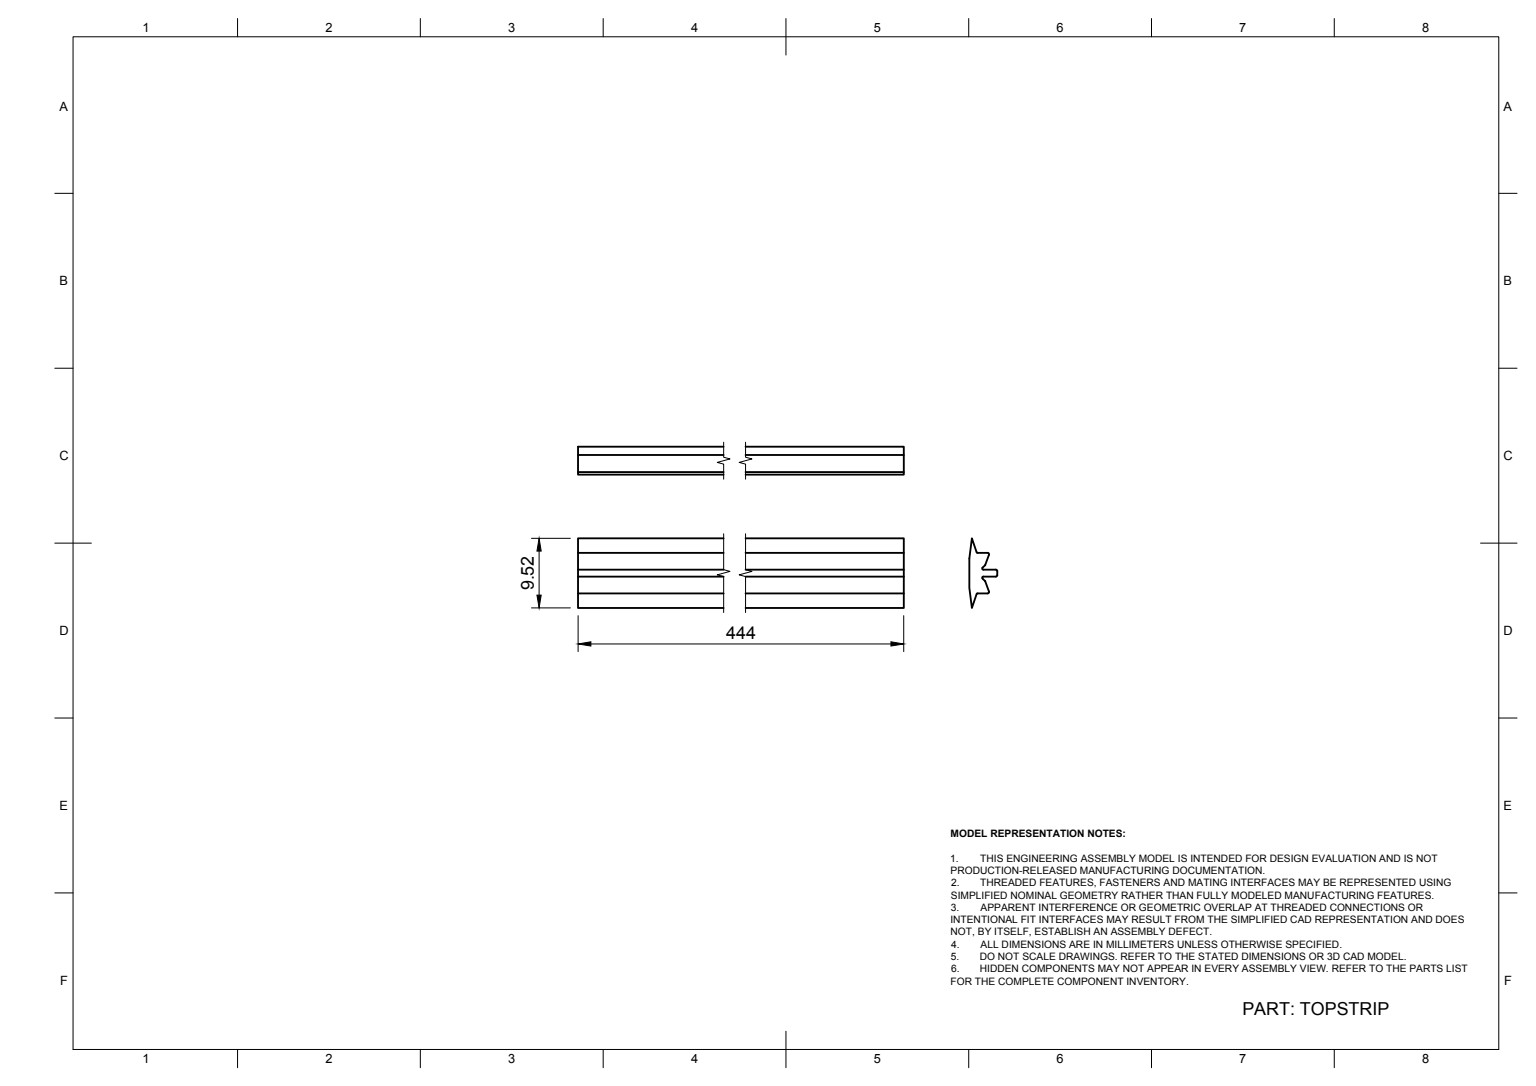
ISO-10303-21;
HEADER;
/* Generated by software containing ST-Developer
 * from STEP Tools, Inc. (www.steptools.com) 
 */

FILE_DESCRIPTION(
/* description */ (''),
/* implementation_level */ '2;1');

FILE_NAME(
/* name */ 'TopStrip.step',
/* time_stamp */ '2026-10-05T11:01:41-07:00',
/* author */ (''),
/* organization */ (''),
/* preprocessor_version */ 'ST-DEVELOPER v20.2',
/* originating_system */ 'Autodesk Translation Framework v15.15.0.0',
/* authorisation */ '');

FILE_SCHEMA (('AUTOMOTIVE_DESIGN { 1 0 10303 214 3 1 1 }'));
ENDSEC;

DATA;
#10=MECHANICAL_DESIGN_GEOMETRIC_PRESENTATION_REPRESENTATION('',(#2137),#215609);
#2119=SHAPE_REPRESENTATION_RELATIONSHIP('SRR','None',#215644,#2128);
#2128=ADVANCED_BREP_SHAPE_REPRESENTATION('',(#2146),#215600);
#2137=STYLED_ITEM('',(#215698),#2146);
#2146=MANIFOLD_SOLID_BREP('Body1',#28080);
#2155=CYLINDRICAL_SURFACE('',#28193,0.127);
#2156=CYLINDRICAL_SURFACE('',#28196,0.202999999999999);
#2157=CYLINDRICAL_SURFACE('',#28199,0.127000000000001);
#2158=CYLINDRICAL_SURFACE('',#28202,0.159000000000001);
#2159=CYLINDRICAL_SURFACE('',#28205,0.203000000000001);
#2160=CYLINDRICAL_SURFACE('',#28209,0.203);
#2161=CYLINDRICAL_SURFACE('',#28212,0.159000000000001);
#2162=CYLINDRICAL_SURFACE('',#28215,0.127000000000001);
#2163=CYLINDRICAL_SURFACE('',#28218,0.203);
#2164=CYLINDRICAL_SURFACE('',#28221,0.126999999999999);
#2964=FACE_OUTER_BOUND('',#4277,.T.);
#2965=FACE_OUTER_BOUND('',#4278,.T.);
#2966=FACE_OUTER_BOUND('',#4279,.T.);
#2967=FACE_OUTER_BOUND('',#4280,.T.);
#2968=FACE_OUTER_BOUND('',#4281,.T.);
#2969=FACE_OUTER_BOUND('',#4282,.T.);
#2970=FACE_OUTER_BOUND('',#4283,.T.);
#2971=FACE_OUTER_BOUND('',#4284,.T.);
#2972=FACE_OUTER_BOUND('',#4285,.T.);
#2973=FACE_OUTER_BOUND('',#4286,.T.);
#2974=FACE_OUTER_BOUND('',#4287,.T.);
#2975=FACE_OUTER_BOUND('',#4288,.T.);
#2976=FACE_OUTER_BOUND('',#4289,.T.);
#2977=FACE_OUTER_BOUND('',#4290,.T.);
#2978=FACE_OUTER_BOUND('',#4291,.T.);
#2979=FACE_OUTER_BOUND('',#4292,.T.);
#2980=FACE_OUTER_BOUND('',#4293,.T.);
#2981=FACE_OUTER_BOUND('',#4294,.T.);
#2982=FACE_OUTER_BOUND('',#4295,.T.);
#2983=FACE_OUTER_BOUND('',#4296,.T.);
#2984=FACE_OUTER_BOUND('',#4297,.T.);
#2985=FACE_OUTER_BOUND('',#4298,.T.);
#2986=FACE_OUTER_BOUND('',#4299,.T.);
#2987=FACE_OUTER_BOUND('',#4300,.T.);
#2988=FACE_OUTER_BOUND('',#4301,.T.);
#2989=FACE_OUTER_BOUND('',#4302,.T.);
#2990=FACE_OUTER_BOUND('',#4303,.T.);
#4277=EDGE_LOOP('',(#17529,#17530,#17531,#17532,#17533,#17534,#17535,#17536,
#17537,#17538,#17539,#17540,#17541,#17542,#17543,#17544,#17545,#17546,#17547,
#17548,#17549,#17550,#17551,#17552,#17553));
#4278=EDGE_LOOP('',(#17554,#17555,#17556,#17557));
#4279=EDGE_LOOP('',(#17558,#17559,#17560,#17561));
#4280=EDGE_LOOP('',(#17562,#17563,#17564,#17565));
#4281=EDGE_LOOP('',(#17566,#17567,#17568,#17569));
#4282=EDGE_LOOP('',(#17570,#17571,#17572,#17573));
#4283=EDGE_LOOP('',(#17574,#17575,#17576,#17577));
#4284=EDGE_LOOP('',(#17578,#17579,#17580,#17581));
#4285=EDGE_LOOP('',(#17582,#17583,#17584,#17585));
#4286=EDGE_LOOP('',(#17586,#17587,#17588,#17589));
#4287=EDGE_LOOP('',(#17590,#17591,#17592,#17593));
#4288=EDGE_LOOP('',(#17594,#17595,#17596,#17597));
#4289=EDGE_LOOP('',(#17598,#17599,#17600,#17601));
#4290=EDGE_LOOP('',(#17602,#17603,#17604,#17605));
#4291=EDGE_LOOP('',(#17606,#17607,#17608,#17609));
#4292=EDGE_LOOP('',(#17610,#17611,#17612,#17613));
#4293=EDGE_LOOP('',(#17614,#17615,#17616,#17617));
#4294=EDGE_LOOP('',(#17618,#17619,#17620,#17621));
#4295=EDGE_LOOP('',(#17622,#17623,#17624,#17625));
#4296=EDGE_LOOP('',(#17626,#17627,#17628,#17629));
#4297=EDGE_LOOP('',(#17630,#17631,#17632,#17633));
#4298=EDGE_LOOP('',(#17634,#17635,#17636,#17637));
#4299=EDGE_LOOP('',(#17638,#17639,#17640,#17641));
#4300=EDGE_LOOP('',(#17642,#17643,#17644,#17645));
#4301=EDGE_LOOP('',(#17646,#17647,#17648,#17649));
#4302=EDGE_LOOP('',(#17650,#17651,#17652,#17653));
#4303=EDGE_LOOP('',(#17654,#17655,#17656,#17657,#17658,#17659,#17660,#17661,
#17662,#17663,#17664,#17665,#17666,#17667,#17668,#17669,#17670,#17671,#17672,
#17673,#17674,#17675,#17676,#17677,#17678));
#5664=CIRCLE('',#28181,0.127);
#5665=CIRCLE('',#28182,0.202999999999999);
#5666=CIRCLE('',#28183,0.127000000000001);
#5667=CIRCLE('',#28184,0.159000000000001);
#5668=CIRCLE('',#28185,0.203000000000001);
#5669=CIRCLE('',#28186,0.203);
#5670=CIRCLE('',#28187,0.159000000000001);
#5671=CIRCLE('',#28188,0.127000000000001);
#5672=CIRCLE('',#28189,0.203);
#5673=CIRCLE('',#28190,0.126999999999999);
#5674=CIRCLE('',#28194,0.127);
#5675=CIRCLE('',#28197,0.202999999999999);
#5676=CIRCLE('',#28200,0.127000000000001);
#5677=CIRCLE('',#28203,0.159000000000001);
#5678=CIRCLE('',#28206,0.203000000000001);
#5679=CIRCLE('',#28210,0.203);
#5680=CIRCLE('',#28213,0.159000000000001);
#5681=CIRCLE('',#28216,0.127000000000001);
#5682=CIRCLE('',#28219,0.203);
#5683=CIRCLE('',#28222,0.126999999999999);
#6296=LINE('',#35986,#8141);
#6297=LINE('',#35988,#8142);
#6298=LINE('',#35990,#8143);
#6299=LINE('',#35994,#8144);
#6300=LINE('',#35998,#8145);
#6301=LINE('',#36002,#8146);
#6302=LINE('',#36006,#8147);
#6303=LINE('',#36010,#8148);
#6304=LINE('',#36012,#8149);
#6305=LINE('',#36016,#8150);
#6306=LINE('',#36020,#8151);
#6307=LINE('',#36024,#8152);
#6308=LINE('',#36028,#8153);
#6309=LINE('',#36032,#8154);
#6310=LINE('',#36033,#8155);
#6311=LINE('',#36036,#8156);
#6312=LINE('',#36038,#8157);
#6313=LINE('',#36039,#8158);
#6314=LINE('',#36042,#8159);
#6315=LINE('',#36043,#8160);
#6316=LINE('',#36047,#8161);
#6317=LINE('',#36050,#8162);
#6318=LINE('',#36051,#8163);
#6319=LINE('',#36055,#8164);
#6320=LINE('',#36058,#8165);
#6321=LINE('',#36059,#8166);
#6322=LINE('',#36063,#8167);
#6323=LINE('',#36066,#8168);
#6324=LINE('',#36067,#8169);
#6325=LINE('',#36071,#8170);
#6326=LINE('',#36074,#8171);
#6327=LINE('',#36075,#8172);
#6328=LINE('',#36079,#8173);
#6329=LINE('',#36082,#8174);
#6330=LINE('',#36083,#8175);
#6331=LINE('',#36086,#8176);
#6332=LINE('',#36087,#8177);
#6333=LINE('',#36091,#8178);
#6334=LINE('',#36094,#8179);
#6335=LINE('',#36095,#8180);
#6336=LINE('',#36099,#8181);
#6337=LINE('',#36102,#8182);
#6338=LINE('',#36103,#8183);
#6339=LINE('',#36107,#8184);
#6340=LINE('',#36110,#8185);
#6341=LINE('',#36111,#8186);
#6342=LINE('',#36115,#8187);
#6343=LINE('',#36118,#8188);
#6344=LINE('',#36119,#8189);
#6345=LINE('',#36123,#8190);
#6346=LINE('',#36126,#8191);
#6347=LINE('',#36127,#8192);
#6348=LINE('',#36130,#8193);
#6349=LINE('',#36131,#8194);
#6350=LINE('',#36133,#8195);
#8141=VECTOR('',#30170,10.);
#8142=VECTOR('',#30171,10.);
#8143=VECTOR('',#30172,10.);
#8144=VECTOR('',#30175,10.);
#8145=VECTOR('',#30178,9.99999999999999);
#8146=VECTOR('',#30181,10.);
#8147=VECTOR('',#30184,10.);
#8148=VECTOR('',#30187,9.99999999999999);
#8149=VECTOR('',#30188,9.99999999999999);
#8150=VECTOR('',#30191,10.);
#8151=VECTOR('',#30194,10.);
#8152=VECTOR('',#30197,9.99999999999999);
#8153=VECTOR('',#30200,10.);
#8154=VECTOR('',#30203,10.);
#8155=VECTOR('',#30204,10.);
#8156=VECTOR('',#30207,10.);
#8157=VECTOR('',#30208,10.);
#8158=VECTOR('',#30209,10.);
#8159=VECTOR('',#30212,10.);
#8160=VECTOR('',#30213,10.);
#8161=VECTOR('',#30218,10.);
#8162=VECTOR('',#30221,10.);
#8163=VECTOR('',#30222,10.);
#8164=VECTOR('',#30227,10.);
#8165=VECTOR('',#30230,9.99999999999999);
#8166=VECTOR('',#30231,10.);
#8167=VECTOR('',#30236,10.);
#8168=VECTOR('',#30239,10.);
#8169=VECTOR('',#30240,10.);
#8170=VECTOR('',#30245,10.);
#8171=VECTOR('',#30248,10.);
#8172=VECTOR('',#30249,10.);
#8173=VECTOR('',#30254,10.);
#8174=VECTOR('',#30257,9.99999999999999);
#8175=VECTOR('',#30258,10.);
#8176=VECTOR('',#30261,9.99999999999999);
#8177=VECTOR('',#30262,10.);
#8178=VECTOR('',#30267,10.);
#8179=VECTOR('',#30270,10.);
#8180=VECTOR('',#30271,10.);
#8181=VECTOR('',#30276,10.);
#8182=VECTOR('',#30279,10.);
#8183=VECTOR('',#30280,10.);
#8184=VECTOR('',#30285,10.);
#8185=VECTOR('',#30288,9.99999999999999);
#8186=VECTOR('',#30289,10.);
#8187=VECTOR('',#30294,10.);
#8188=VECTOR('',#30297,10.);
#8189=VECTOR('',#30298,10.);
#8190=VECTOR('',#30303,10.);
#8191=VECTOR('',#30306,10.);
#8192=VECTOR('',#30307,10.);
#8193=VECTOR('',#30310,10.);
#8194=VECTOR('',#30311,10.);
#8195=VECTOR('',#30314,10.);
#9986=VERTEX_POINT('',#35984);
#9987=VERTEX_POINT('',#35985);
#9988=VERTEX_POINT('',#35987);
#9989=VERTEX_POINT('',#35989);
#9990=VERTEX_POINT('',#35991);
#9991=VERTEX_POINT('',#35993);
#9992=VERTEX_POINT('',#35995);
#9993=VERTEX_POINT('',#35997);
#9994=VERTEX_POINT('',#35999);
#9995=VERTEX_POINT('',#36001);
#9996=VERTEX_POINT('',#36003);
#9997=VERTEX_POINT('',#36005);
#9998=VERTEX_POINT('',#36007);
#9999=VERTEX_POINT('',#36009);
#10000=VERTEX_POINT('',#36011);
#10001=VERTEX_POINT('',#36013);
#10002=VERTEX_POINT('',#36015);
#10003=VERTEX_POINT('',#36017);
#10004=VERTEX_POINT('',#36019);
#10005=VERTEX_POINT('',#36021);
#10006=VERTEX_POINT('',#36023);
#10007=VERTEX_POINT('',#36025);
#10008=VERTEX_POINT('',#36027);
#10009=VERTEX_POINT('',#36029);
#10010=VERTEX_POINT('',#36031);
#10011=VERTEX_POINT('',#36035);
#10012=VERTEX_POINT('',#36037);
#10013=VERTEX_POINT('',#36041);
#10014=VERTEX_POINT('',#36045);
#10015=VERTEX_POINT('',#36049);
#10016=VERTEX_POINT('',#36053);
#10017=VERTEX_POINT('',#36057);
#10018=VERTEX_POINT('',#36061);
#10019=VERTEX_POINT('',#36065);
#10020=VERTEX_POINT('',#36069);
#10021=VERTEX_POINT('',#36073);
#10022=VERTEX_POINT('',#36077);
#10023=VERTEX_POINT('',#36081);
#10024=VERTEX_POINT('',#36085);
#10025=VERTEX_POINT('',#36089);
#10026=VERTEX_POINT('',#36093);
#10027=VERTEX_POINT('',#36097);
#10028=VERTEX_POINT('',#36101);
#10029=VERTEX_POINT('',#36105);
#10030=VERTEX_POINT('',#36109);
#10031=VERTEX_POINT('',#36113);
#10032=VERTEX_POINT('',#36117);
#10033=VERTEX_POINT('',#36121);
#10034=VERTEX_POINT('',#36125);
#10035=VERTEX_POINT('',#36129);
#13126=EDGE_CURVE('',#9986,#9987,#6296,.T.);
#13127=EDGE_CURVE('',#9987,#9988,#6297,.T.);
#13128=EDGE_CURVE('',#9988,#9989,#6298,.T.);
#13129=EDGE_CURVE('',#9989,#9990,#5664,.T.);
#13130=EDGE_CURVE('',#9990,#9991,#6299,.T.);
#13131=EDGE_CURVE('',#9991,#9992,#5665,.T.);
#13132=EDGE_CURVE('',#9992,#9993,#6300,.T.);
#13133=EDGE_CURVE('',#9993,#9994,#5666,.T.);
#13134=EDGE_CURVE('',#9994,#9995,#6301,.T.);
#13135=EDGE_CURVE('',#9995,#9996,#5667,.T.);
#13136=EDGE_CURVE('',#9996,#9997,#6302,.T.);
#13137=EDGE_CURVE('',#9997,#9998,#5668,.T.);
#13138=EDGE_CURVE('',#9998,#9999,#6303,.T.);
#13139=EDGE_CURVE('',#9999,#10000,#6304,.T.);
#13140=EDGE_CURVE('',#10000,#10001,#5669,.T.);
#13141=EDGE_CURVE('',#10001,#10002,#6305,.T.);
#13142=EDGE_CURVE('',#10002,#10003,#5670,.T.);
#13143=EDGE_CURVE('',#10003,#10004,#6306,.T.);
#13144=EDGE_CURVE('',#10004,#10005,#5671,.T.);
#13145=EDGE_CURVE('',#10005,#10006,#6307,.T.);
#13146=EDGE_CURVE('',#10006,#10007,#5672,.T.);
#13147=EDGE_CURVE('',#10007,#10008,#6308,.T.);
#13148=EDGE_CURVE('',#10008,#10009,#5673,.T.);
#13149=EDGE_CURVE('',#10009,#10010,#6309,.T.);
#13150=EDGE_CURVE('',#10010,#9986,#6310,.T.);
#13151=EDGE_CURVE('',#10011,#9987,#6311,.T.);
#13152=EDGE_CURVE('',#10012,#10011,#6312,.T.);
#13153=EDGE_CURVE('',#9988,#10012,#6313,.T.);
#13154=EDGE_CURVE('',#10013,#10012,#6314,.T.);
#13155=EDGE_CURVE('',#9989,#10013,#6315,.T.);
#13156=EDGE_CURVE('',#10014,#10013,#5674,.T.);
#13157=EDGE_CURVE('',#9990,#10014,#6316,.T.);
#13158=EDGE_CURVE('',#10015,#10014,#6317,.T.);
#13159=EDGE_CURVE('',#9991,#10015,#6318,.T.);
#13160=EDGE_CURVE('',#10016,#10015,#5675,.T.);
#13161=EDGE_CURVE('',#9992,#10016,#6319,.T.);
#13162=EDGE_CURVE('',#10017,#10016,#6320,.T.);
#13163=EDGE_CURVE('',#9993,#10017,#6321,.T.);
#13164=EDGE_CURVE('',#10018,#10017,#5676,.T.);
#13165=EDGE_CURVE('',#9994,#10018,#6322,.T.);
#13166=EDGE_CURVE('',#10019,#10018,#6323,.T.);
#13167=EDGE_CURVE('',#9995,#10019,#6324,.T.);
#13168=EDGE_CURVE('',#10020,#10019,#5677,.T.);
#13169=EDGE_CURVE('',#9996,#10020,#6325,.T.);
#13170=EDGE_CURVE('',#10021,#10020,#6326,.T.);
#13171=EDGE_CURVE('',#9997,#10021,#6327,.T.);
#13172=EDGE_CURVE('',#10022,#10021,#5678,.T.);
#13173=EDGE_CURVE('',#9998,#10022,#6328,.T.);
#13174=EDGE_CURVE('',#10023,#10022,#6329,.T.);
#13175=EDGE_CURVE('',#9999,#10023,#6330,.T.);
#13176=EDGE_CURVE('',#10024,#10023,#6331,.T.);
#13177=EDGE_CURVE('',#10000,#10024,#6332,.T.);
#13178=EDGE_CURVE('',#10025,#10024,#5679,.T.);
#13179=EDGE_CURVE('',#10001,#10025,#6333,.T.);
#13180=EDGE_CURVE('',#10026,#10025,#6334,.T.);
#13181=EDGE_CURVE('',#10002,#10026,#6335,.T.);
#13182=EDGE_CURVE('',#10027,#10026,#5680,.T.);
#13183=EDGE_CURVE('',#10003,#10027,#6336,.T.);
#13184=EDGE_CURVE('',#10028,#10027,#6337,.T.);
#13185=EDGE_CURVE('',#10004,#10028,#6338,.T.);
#13186=EDGE_CURVE('',#10029,#10028,#5681,.T.);
#13187=EDGE_CURVE('',#10005,#10029,#6339,.T.);
#13188=EDGE_CURVE('',#10030,#10029,#6340,.T.);
#13189=EDGE_CURVE('',#10006,#10030,#6341,.T.);
#13190=EDGE_CURVE('',#10031,#10030,#5682,.T.);
#13191=EDGE_CURVE('',#10007,#10031,#6342,.T.);
#13192=EDGE_CURVE('',#10032,#10031,#6343,.T.);
#13193=EDGE_CURVE('',#10008,#10032,#6344,.T.);
#13194=EDGE_CURVE('',#10033,#10032,#5683,.T.);
#13195=EDGE_CURVE('',#10009,#10033,#6345,.T.);
#13196=EDGE_CURVE('',#10034,#10033,#6346,.T.);
#13197=EDGE_CURVE('',#10010,#10034,#6347,.T.);
#13198=EDGE_CURVE('',#10035,#10034,#6348,.T.);
#13199=EDGE_CURVE('',#9986,#10035,#6349,.T.);
#13200=EDGE_CURVE('',#10011,#10035,#6350,.T.);
#17529=ORIENTED_EDGE('',*,*,#13126,.T.);
#17530=ORIENTED_EDGE('',*,*,#13127,.T.);
#17531=ORIENTED_EDGE('',*,*,#13128,.T.);
#17532=ORIENTED_EDGE('',*,*,#13129,.T.);
#17533=ORIENTED_EDGE('',*,*,#13130,.T.);
#17534=ORIENTED_EDGE('',*,*,#13131,.T.);
#17535=ORIENTED_EDGE('',*,*,#13132,.T.);
#17536=ORIENTED_EDGE('',*,*,#13133,.T.);
#17537=ORIENTED_EDGE('',*,*,#13134,.T.);
#17538=ORIENTED_EDGE('',*,*,#13135,.T.);
#17539=ORIENTED_EDGE('',*,*,#13136,.T.);
#17540=ORIENTED_EDGE('',*,*,#13137,.T.);
#17541=ORIENTED_EDGE('',*,*,#13138,.T.);
#17542=ORIENTED_EDGE('',*,*,#13139,.T.);
#17543=ORIENTED_EDGE('',*,*,#13140,.T.);
#17544=ORIENTED_EDGE('',*,*,#13141,.T.);
#17545=ORIENTED_EDGE('',*,*,#13142,.T.);
#17546=ORIENTED_EDGE('',*,*,#13143,.T.);
#17547=ORIENTED_EDGE('',*,*,#13144,.T.);
#17548=ORIENTED_EDGE('',*,*,#13145,.T.);
#17549=ORIENTED_EDGE('',*,*,#13146,.T.);
#17550=ORIENTED_EDGE('',*,*,#13147,.T.);
#17551=ORIENTED_EDGE('',*,*,#13148,.T.);
#17552=ORIENTED_EDGE('',*,*,#13149,.T.);
#17553=ORIENTED_EDGE('',*,*,#13150,.T.);
#17554=ORIENTED_EDGE('',*,*,#13151,.F.);
#17555=ORIENTED_EDGE('',*,*,#13152,.F.);
#17556=ORIENTED_EDGE('',*,*,#13153,.F.);
#17557=ORIENTED_EDGE('',*,*,#13127,.F.);
#17558=ORIENTED_EDGE('',*,*,#13153,.T.);
#17559=ORIENTED_EDGE('',*,*,#13154,.F.);
#17560=ORIENTED_EDGE('',*,*,#13155,.F.);
#17561=ORIENTED_EDGE('',*,*,#13128,.F.);
#17562=ORIENTED_EDGE('',*,*,#13155,.T.);
#17563=ORIENTED_EDGE('',*,*,#13156,.F.);
#17564=ORIENTED_EDGE('',*,*,#13157,.F.);
#17565=ORIENTED_EDGE('',*,*,#13129,.F.);
#17566=ORIENTED_EDGE('',*,*,#13157,.T.);
#17567=ORIENTED_EDGE('',*,*,#13158,.F.);
#17568=ORIENTED_EDGE('',*,*,#13159,.F.);
#17569=ORIENTED_EDGE('',*,*,#13130,.F.);
#17570=ORIENTED_EDGE('',*,*,#13159,.T.);
#17571=ORIENTED_EDGE('',*,*,#13160,.F.);
#17572=ORIENTED_EDGE('',*,*,#13161,.F.);
#17573=ORIENTED_EDGE('',*,*,#13131,.F.);
#17574=ORIENTED_EDGE('',*,*,#13161,.T.);
#17575=ORIENTED_EDGE('',*,*,#13162,.F.);
#17576=ORIENTED_EDGE('',*,*,#13163,.F.);
#17577=ORIENTED_EDGE('',*,*,#13132,.F.);
#17578=ORIENTED_EDGE('',*,*,#13163,.T.);
#17579=ORIENTED_EDGE('',*,*,#13164,.F.);
#17580=ORIENTED_EDGE('',*,*,#13165,.F.);
#17581=ORIENTED_EDGE('',*,*,#13133,.F.);
#17582=ORIENTED_EDGE('',*,*,#13165,.T.);
#17583=ORIENTED_EDGE('',*,*,#13166,.F.);
#17584=ORIENTED_EDGE('',*,*,#13167,.F.);
#17585=ORIENTED_EDGE('',*,*,#13134,.F.);
#17586=ORIENTED_EDGE('',*,*,#13167,.T.);
#17587=ORIENTED_EDGE('',*,*,#13168,.F.);
#17588=ORIENTED_EDGE('',*,*,#13169,.F.);
#17589=ORIENTED_EDGE('',*,*,#13135,.F.);
#17590=ORIENTED_EDGE('',*,*,#13169,.T.);
#17591=ORIENTED_EDGE('',*,*,#13170,.F.);
#17592=ORIENTED_EDGE('',*,*,#13171,.F.);
#17593=ORIENTED_EDGE('',*,*,#13136,.F.);
#17594=ORIENTED_EDGE('',*,*,#13171,.T.);
#17595=ORIENTED_EDGE('',*,*,#13172,.F.);
#17596=ORIENTED_EDGE('',*,*,#13173,.F.);
#17597=ORIENTED_EDGE('',*,*,#13137,.F.);
#17598=ORIENTED_EDGE('',*,*,#13173,.T.);
#17599=ORIENTED_EDGE('',*,*,#13174,.F.);
#17600=ORIENTED_EDGE('',*,*,#13175,.F.);
#17601=ORIENTED_EDGE('',*,*,#13138,.F.);
#17602=ORIENTED_EDGE('',*,*,#13175,.T.);
#17603=ORIENTED_EDGE('',*,*,#13176,.F.);
#17604=ORIENTED_EDGE('',*,*,#13177,.F.);
#17605=ORIENTED_EDGE('',*,*,#13139,.F.);
#17606=ORIENTED_EDGE('',*,*,#13177,.T.);
#17607=ORIENTED_EDGE('',*,*,#13178,.F.);
#17608=ORIENTED_EDGE('',*,*,#13179,.F.);
#17609=ORIENTED_EDGE('',*,*,#13140,.F.);
#17610=ORIENTED_EDGE('',*,*,#13179,.T.);
#17611=ORIENTED_EDGE('',*,*,#13180,.F.);
#17612=ORIENTED_EDGE('',*,*,#13181,.F.);
#17613=ORIENTED_EDGE('',*,*,#13141,.F.);
#17614=ORIENTED_EDGE('',*,*,#13181,.T.);
#17615=ORIENTED_EDGE('',*,*,#13182,.F.);
#17616=ORIENTED_EDGE('',*,*,#13183,.F.);
#17617=ORIENTED_EDGE('',*,*,#13142,.F.);
#17618=ORIENTED_EDGE('',*,*,#13183,.T.);
#17619=ORIENTED_EDGE('',*,*,#13184,.F.);
#17620=ORIENTED_EDGE('',*,*,#13185,.F.);
#17621=ORIENTED_EDGE('',*,*,#13143,.F.);
#17622=ORIENTED_EDGE('',*,*,#13185,.T.);
#17623=ORIENTED_EDGE('',*,*,#13186,.F.);
#17624=ORIENTED_EDGE('',*,*,#13187,.F.);
#17625=ORIENTED_EDGE('',*,*,#13144,.F.);
#17626=ORIENTED_EDGE('',*,*,#13187,.T.);
#17627=ORIENTED_EDGE('',*,*,#13188,.F.);
#17628=ORIENTED_EDGE('',*,*,#13189,.F.);
#17629=ORIENTED_EDGE('',*,*,#13145,.F.);
#17630=ORIENTED_EDGE('',*,*,#13189,.T.);
#17631=ORIENTED_EDGE('',*,*,#13190,.F.);
#17632=ORIENTED_EDGE('',*,*,#13191,.F.);
#17633=ORIENTED_EDGE('',*,*,#13146,.F.);
#17634=ORIENTED_EDGE('',*,*,#13191,.T.);
#17635=ORIENTED_EDGE('',*,*,#13192,.F.);
#17636=ORIENTED_EDGE('',*,*,#13193,.F.);
#17637=ORIENTED_EDGE('',*,*,#13147,.F.);
#17638=ORIENTED_EDGE('',*,*,#13193,.T.);
#17639=ORIENTED_EDGE('',*,*,#13194,.F.);
#17640=ORIENTED_EDGE('',*,*,#13195,.F.);
#17641=ORIENTED_EDGE('',*,*,#13148,.F.);
#17642=ORIENTED_EDGE('',*,*,#13195,.T.);
#17643=ORIENTED_EDGE('',*,*,#13196,.F.);
#17644=ORIENTED_EDGE('',*,*,#13197,.F.);
#17645=ORIENTED_EDGE('',*,*,#13149,.F.);
#17646=ORIENTED_EDGE('',*,*,#13197,.T.);
#17647=ORIENTED_EDGE('',*,*,#13198,.F.);
#17648=ORIENTED_EDGE('',*,*,#13199,.F.);
#17649=ORIENTED_EDGE('',*,*,#13150,.F.);
#17650=ORIENTED_EDGE('',*,*,#13199,.T.);
#17651=ORIENTED_EDGE('',*,*,#13200,.F.);
#17652=ORIENTED_EDGE('',*,*,#13151,.T.);
#17653=ORIENTED_EDGE('',*,*,#13126,.F.);
#17654=ORIENTED_EDGE('',*,*,#13200,.T.);
#17655=ORIENTED_EDGE('',*,*,#13198,.T.);
#17656=ORIENTED_EDGE('',*,*,#13196,.T.);
#17657=ORIENTED_EDGE('',*,*,#13194,.T.);
#17658=ORIENTED_EDGE('',*,*,#13192,.T.);
#17659=ORIENTED_EDGE('',*,*,#13190,.T.);
#17660=ORIENTED_EDGE('',*,*,#13188,.T.);
#17661=ORIENTED_EDGE('',*,*,#13186,.T.);
#17662=ORIENTED_EDGE('',*,*,#13184,.T.);
#17663=ORIENTED_EDGE('',*,*,#13182,.T.);
#17664=ORIENTED_EDGE('',*,*,#13180,.T.);
#17665=ORIENTED_EDGE('',*,*,#13178,.T.);
#17666=ORIENTED_EDGE('',*,*,#13176,.T.);
#17667=ORIENTED_EDGE('',*,*,#13174,.T.);
#17668=ORIENTED_EDGE('',*,*,#13172,.T.);
#17669=ORIENTED_EDGE('',*,*,#13170,.T.);
#17670=ORIENTED_EDGE('',*,*,#13168,.T.);
#17671=ORIENTED_EDGE('',*,*,#13166,.T.);
#17672=ORIENTED_EDGE('',*,*,#13164,.T.);
#17673=ORIENTED_EDGE('',*,*,#13162,.T.);
#17674=ORIENTED_EDGE('',*,*,#13160,.T.);
#17675=ORIENTED_EDGE('',*,*,#13158,.T.);
#17676=ORIENTED_EDGE('',*,*,#13156,.T.);
#17677=ORIENTED_EDGE('',*,*,#13154,.T.);
#17678=ORIENTED_EDGE('',*,*,#13152,.T.);
#26335=PLANE('',#28180);
#26336=PLANE('',#28191);
#26337=PLANE('',#28192);
#26338=PLANE('',#28195);
#26339=PLANE('',#28198);
#26340=PLANE('',#28201);
#26341=PLANE('',#28204);
#26342=PLANE('',#28207);
#26343=PLANE('',#28208);
#26344=PLANE('',#28211);
#26345=PLANE('',#28214);
#26346=PLANE('',#28217);
#26347=PLANE('',#28220);
#26348=PLANE('',#28223);
#26349=PLANE('',#28224);
#26350=PLANE('',#28225);
#26351=PLANE('',#28226);
#26767=ADVANCED_FACE('',(#2964),#26335,.F.);
#26768=ADVANCED_FACE('',(#2965),#26336,.T.);
#26769=ADVANCED_FACE('',(#2966),#26337,.T.);
#26770=ADVANCED_FACE('',(#2967),#2155,.F.);
#26771=ADVANCED_FACE('',(#2968),#26338,.T.);
#26772=ADVANCED_FACE('',(#2969),#2156,.T.);
#26773=ADVANCED_FACE('',(#2970),#26339,.T.);
#26774=ADVANCED_FACE('',(#2971),#2157,.T.);
#26775=ADVANCED_FACE('',(#2972),#26340,.T.);
#26776=ADVANCED_FACE('',(#2973),#2158,.F.);
#26777=ADVANCED_FACE('',(#2974),#26341,.T.);
#26778=ADVANCED_FACE('',(#2975),#2159,.T.);
#26779=ADVANCED_FACE('',(#2976),#26342,.T.);
#26780=ADVANCED_FACE('',(#2977),#26343,.T.);
#26781=ADVANCED_FACE('',(#2978),#2160,.T.);
#26782=ADVANCED_FACE('',(#2979),#26344,.T.);
#26783=ADVANCED_FACE('',(#2980),#2161,.F.);
#26784=ADVANCED_FACE('',(#2981),#26345,.T.);
#26785=ADVANCED_FACE('',(#2982),#2162,.T.);
#26786=ADVANCED_FACE('',(#2983),#26346,.T.);
#26787=ADVANCED_FACE('',(#2984),#2163,.T.);
#26788=ADVANCED_FACE('',(#2985),#26347,.T.);
#26789=ADVANCED_FACE('',(#2986),#2164,.F.);
#26790=ADVANCED_FACE('',(#2987),#26348,.T.);
#26791=ADVANCED_FACE('',(#2988),#26349,.T.);
#26792=ADVANCED_FACE('',(#2989),#26350,.T.);
#26793=ADVANCED_FACE('',(#2990),#26351,.T.);
#28080=CLOSED_SHELL('',(#26767,#26768,#26769,#26770,#26771,#26772,#26773,
#26774,#26775,#26776,#26777,#26778,#26779,#26780,#26781,#26782,#26783,#26784,
#26785,#26786,#26787,#26788,#26789,#26790,#26791,#26792,#26793));
#28179=AXIS2_PLACEMENT_3D('',#35982,#30166,#30167);
#28180=AXIS2_PLACEMENT_3D('',#35983,#30168,#30169);
#28181=AXIS2_PLACEMENT_3D('',#35992,#30173,#30174);
#28182=AXIS2_PLACEMENT_3D('',#35996,#30176,#30177);
#28183=AXIS2_PLACEMENT_3D('',#36000,#30179,#30180);
#28184=AXIS2_PLACEMENT_3D('',#36004,#30182,#30183);
#28185=AXIS2_PLACEMENT_3D('',#36008,#30185,#30186);
#28186=AXIS2_PLACEMENT_3D('',#36014,#30189,#30190);
#28187=AXIS2_PLACEMENT_3D('',#36018,#30192,#30193);
#28188=AXIS2_PLACEMENT_3D('',#36022,#30195,#30196);
#28189=AXIS2_PLACEMENT_3D('',#36026,#30198,#30199);
#28190=AXIS2_PLACEMENT_3D('',#36030,#30201,#30202);
#28191=AXIS2_PLACEMENT_3D('',#36034,#30205,#30206);
#28192=AXIS2_PLACEMENT_3D('',#36040,#30210,#30211);
#28193=AXIS2_PLACEMENT_3D('',#36044,#30214,#30215);
#28194=AXIS2_PLACEMENT_3D('',#36046,#30216,#30217);
#28195=AXIS2_PLACEMENT_3D('',#36048,#30219,#30220);
#28196=AXIS2_PLACEMENT_3D('',#36052,#30223,#30224);
#28197=AXIS2_PLACEMENT_3D('',#36054,#30225,#30226);
#28198=AXIS2_PLACEMENT_3D('',#36056,#30228,#30229);
#28199=AXIS2_PLACEMENT_3D('',#36060,#30232,#30233);
#28200=AXIS2_PLACEMENT_3D('',#36062,#30234,#30235);
#28201=AXIS2_PLACEMENT_3D('',#36064,#30237,#30238);
#28202=AXIS2_PLACEMENT_3D('',#36068,#30241,#30242);
#28203=AXIS2_PLACEMENT_3D('',#36070,#30243,#30244);
#28204=AXIS2_PLACEMENT_3D('',#36072,#30246,#30247);
#28205=AXIS2_PLACEMENT_3D('',#36076,#30250,#30251);
#28206=AXIS2_PLACEMENT_3D('',#36078,#30252,#30253);
#28207=AXIS2_PLACEMENT_3D('',#36080,#30255,#30256);
#28208=AXIS2_PLACEMENT_3D('',#36084,#30259,#30260);
#28209=AXIS2_PLACEMENT_3D('',#36088,#30263,#30264);
#28210=AXIS2_PLACEMENT_3D('',#36090,#30265,#30266);
#28211=AXIS2_PLACEMENT_3D('',#36092,#30268,#30269);
#28212=AXIS2_PLACEMENT_3D('',#36096,#30272,#30273);
#28213=AXIS2_PLACEMENT_3D('',#36098,#30274,#30275);
#28214=AXIS2_PLACEMENT_3D('',#36100,#30277,#30278);
#28215=AXIS2_PLACEMENT_3D('',#36104,#30281,#30282);
#28216=AXIS2_PLACEMENT_3D('',#36106,#30283,#30284);
#28217=AXIS2_PLACEMENT_3D('',#36108,#30286,#30287);
#28218=AXIS2_PLACEMENT_3D('',#36112,#30290,#30291);
#28219=AXIS2_PLACEMENT_3D('',#36114,#30292,#30293);
#28220=AXIS2_PLACEMENT_3D('',#36116,#30295,#30296);
#28221=AXIS2_PLACEMENT_3D('',#36120,#30299,#30300);
#28222=AXIS2_PLACEMENT_3D('',#36122,#30301,#30302);
#28223=AXIS2_PLACEMENT_3D('',#36124,#30304,#30305);
#28224=AXIS2_PLACEMENT_3D('',#36128,#30308,#30309);
#28225=AXIS2_PLACEMENT_3D('',#36132,#30312,#30313);
#28226=AXIS2_PLACEMENT_3D('',#36134,#30315,#30316);
#30166=DIRECTION('axis',(0.,0.,1.));
#30167=DIRECTION('refdir',(1.,0.,0.));
#30168=DIRECTION('center_axis',(0.,0.,1.));
#30169=DIRECTION('ref_axis',(1.,0.,0.));
#30170=DIRECTION('',(-1.,0.,0.));
#30171=DIRECTION('',(-0.992331937885489,0.123601476740492,0.));
#30172=DIRECTION('',(0.947210277746029,0.320612990585676,0.));
#30173=DIRECTION('center_axis',(0.,0.,1.));
#30174=DIRECTION('ref_axis',(0.320612990585677,-0.947210277746029,0.));
#30175=DIRECTION('',(-0.000226892800803133,0.999999974259828,0.));
#30176=DIRECTION('center_axis',(0.,0.,-1.));
#30177=DIRECTION('ref_axis',(0.341806925031389,0.939770198506308,0.));
#30178=DIRECTION('',(0.939770198506308,-0.341806925031389,0.));
#30179=DIRECTION('center_axis',(0.,0.,-1.));
#30180=DIRECTION('ref_axis',(0.721603167216852,0.692306918254186,0.));
#30181=DIRECTION('',(0.692306918254186,-0.721603167216852,0.));
#30182=DIRECTION('center_axis',(0.,0.,1.));
#30183=DIRECTION('ref_axis',(-0.721603167216849,-0.692306918254189,0.));
#30184=DIRECTION('',(-0.000226892800815894,0.999999974259828,0.));
#30185=DIRECTION('center_axis',(0.,0.,-1.));
#30186=DIRECTION('ref_axis',(-0.000226892800814663,0.999999974259828,0.));
#30187=DIRECTION('',(0.999991534671702,0.00411467920174865,0.));
#30188=DIRECTION('',(0.999991534671702,-0.00411467920174865,0.));
#30189=DIRECTION('center_axis',(0.,0.,-1.));
#30190=DIRECTION('ref_axis',(0.999999974259828,-0.000226892800814664,0.));
#30191=DIRECTION('',(-0.000226892800815894,-0.999999974259828,0.));
#30192=DIRECTION('center_axis',(0.,0.,1.));
#30193=DIRECTION('ref_axis',(-0.999999974259828,0.000226892800815902,0.));
#30194=DIRECTION('',(0.692306918254186,0.721603167216852,0.));
#30195=DIRECTION('center_axis',(0.,0.,-1.));
#30196=DIRECTION('ref_axis',(-0.341806925031389,0.939770198506308,0.));
#30197=DIRECTION('',(0.939770198506308,0.341806925031389,0.));
#30198=DIRECTION('center_axis',(0.,0.,-1.));
#30199=DIRECTION('ref_axis',(0.999999974259828,-0.000226892800803726,0.));
#30200=DIRECTION('',(-0.000226892800803133,-0.999999974259828,0.));
#30201=DIRECTION('center_axis',(0.,0.,1.));
#30202=DIRECTION('ref_axis',(-0.999999974259828,0.000226892800803038,0.));
#30203=DIRECTION('',(0.947210277746029,-0.320612990585676,0.));
#30204=DIRECTION('',(-0.992331937885489,-0.123601476740492,0.));
#30205=DIRECTION('center_axis',(-0.123601476740492,-0.992331937885489,0.));
#30206=DIRECTION('ref_axis',(0.992331937885489,-0.123601476740492,0.));
#30207=DIRECTION('',(0.,0.,-1.));
#30208=DIRECTION('',(0.992331937885489,-0.123601476740492,0.));
#30209=DIRECTION('',(0.,0.,1.));
#30210=DIRECTION('center_axis',(-0.320612990585676,0.947210277746029,0.));
#30211=DIRECTION('ref_axis',(-0.947210277746029,-0.320612990585676,0.));
#30212=DIRECTION('',(-0.947210277746029,-0.320612990585676,0.));
#30213=DIRECTION('',(0.,0.,1.));
#30214=DIRECTION('center_axis',(0.,0.,1.));
#30215=DIRECTION('ref_axis',(0.320612990585677,-0.947210277746029,0.));
#30216=DIRECTION('center_axis',(0.,0.,-1.));
#30217=DIRECTION('ref_axis',(0.320612990585677,-0.947210277746029,0.));
#30218=DIRECTION('',(0.,0.,1.));
#30219=DIRECTION('center_axis',(-0.999999974259828,-0.000226892800803133,
0.));
#30220=DIRECTION('ref_axis',(0.000226892800803133,-0.999999974259828,0.));
#30221=DIRECTION('',(0.000226892800803133,-0.999999974259828,0.));
#30222=DIRECTION('',(0.,0.,1.));
#30223=DIRECTION('center_axis',(0.,0.,1.));
#30224=DIRECTION('ref_axis',(0.341806925031389,0.939770198506308,0.));
#30225=DIRECTION('center_axis',(0.,0.,1.));
#30226=DIRECTION('ref_axis',(0.341806925031389,0.939770198506308,0.));
#30227=DIRECTION('',(0.,0.,1.));
#30228=DIRECTION('center_axis',(0.341806925031389,0.939770198506309,0.));
#30229=DIRECTION('ref_axis',(-0.939770198506308,0.341806925031389,0.));
#30230=DIRECTION('',(-0.939770198506308,0.341806925031389,0.));
#30231=DIRECTION('',(0.,0.,1.));
#30232=DIRECTION('center_axis',(0.,0.,1.));
#30233=DIRECTION('ref_axis',(0.721603167216852,0.692306918254186,0.));
#30234=DIRECTION('center_axis',(0.,0.,1.));
#30235=DIRECTION('ref_axis',(0.721603167216852,0.692306918254186,0.));
#30236=DIRECTION('',(0.,0.,1.));
#30237=DIRECTION('center_axis',(0.721603167216852,0.692306918254186,0.));
#30238=DIRECTION('ref_axis',(-0.692306918254186,0.721603167216852,0.));
#30239=DIRECTION('',(-0.692306918254186,0.721603167216852,0.));
#30240=DIRECTION('',(0.,0.,1.));
#30241=DIRECTION('center_axis',(0.,0.,1.));
#30242=DIRECTION('ref_axis',(-0.721603167216849,-0.692306918254189,0.));
#30243=DIRECTION('center_axis',(0.,0.,-1.));
#30244=DIRECTION('ref_axis',(-0.721603167216849,-0.692306918254189,0.));
#30245=DIRECTION('',(0.,0.,1.));
#30246=DIRECTION('center_axis',(-0.999999974259828,-0.000226892800815894,
0.));
#30247=DIRECTION('ref_axis',(0.000226892800815894,-0.999999974259828,0.));
#30248=DIRECTION('',(0.000226892800815894,-0.999999974259828,0.));
#30249=DIRECTION('',(0.,0.,1.));
#30250=DIRECTION('center_axis',(0.,0.,1.));
#30251=DIRECTION('ref_axis',(-0.000226892800814663,0.999999974259828,0.));
#30252=DIRECTION('center_axis',(0.,0.,1.));
#30253=DIRECTION('ref_axis',(-0.000226892800814663,0.999999974259828,0.));
#30254=DIRECTION('',(0.,0.,1.));
#30255=DIRECTION('center_axis',(-0.00411467920174865,0.999991534671702,
0.));
#30256=DIRECTION('ref_axis',(-0.999991534671703,-0.00411467920174865,0.));
#30257=DIRECTION('',(-0.999991534671702,-0.00411467920174865,0.));
#30258=DIRECTION('',(0.,0.,1.));
#30259=DIRECTION('center_axis',(0.00411467920174865,0.999991534671702,0.));
#30260=DIRECTION('ref_axis',(-0.999991534671703,0.00411467920174865,0.));
#30261=DIRECTION('',(-0.999991534671702,0.00411467920174865,0.));
#30262=DIRECTION('',(0.,0.,1.));
#30263=DIRECTION('center_axis',(0.,0.,1.));
#30264=DIRECTION('ref_axis',(0.999999974259828,-0.000226892800814664,0.));
#30265=DIRECTION('center_axis',(0.,0.,1.));
#30266=DIRECTION('ref_axis',(0.999999974259828,-0.000226892800814664,0.));
#30267=DIRECTION('',(0.,0.,1.));
#30268=DIRECTION('center_axis',(0.999999974259828,-0.000226892800815894,
0.));
#30269=DIRECTION('ref_axis',(0.000226892800815894,0.999999974259828,0.));
#30270=DIRECTION('',(0.000226892800815894,0.999999974259828,0.));
#30271=DIRECTION('',(0.,0.,1.));
#30272=DIRECTION('center_axis',(0.,0.,1.));
#30273=DIRECTION('ref_axis',(-0.999999974259828,0.000226892800815902,0.));
#30274=DIRECTION('center_axis',(0.,0.,-1.));
#30275=DIRECTION('ref_axis',(-0.999999974259828,0.000226892800815902,0.));
#30276=DIRECTION('',(0.,0.,1.));
#30277=DIRECTION('center_axis',(-0.721603167216852,0.692306918254186,0.));
#30278=DIRECTION('ref_axis',(-0.692306918254186,-0.721603167216852,0.));
#30279=DIRECTION('',(-0.692306918254186,-0.721603167216852,0.));
#30280=DIRECTION('',(0.,0.,1.));
#30281=DIRECTION('center_axis',(0.,0.,1.));
#30282=DIRECTION('ref_axis',(-0.341806925031389,0.939770198506308,0.));
#30283=DIRECTION('center_axis',(0.,0.,1.));
#30284=DIRECTION('ref_axis',(-0.341806925031389,0.939770198506308,0.));
#30285=DIRECTION('',(0.,0.,1.));
#30286=DIRECTION('center_axis',(-0.341806925031389,0.939770198506309,0.));
#30287=DIRECTION('ref_axis',(-0.939770198506308,-0.341806925031389,0.));
#30288=DIRECTION('',(-0.939770198506308,-0.341806925031389,0.));
#30289=DIRECTION('',(0.,0.,1.));
#30290=DIRECTION('center_axis',(0.,0.,1.));
#30291=DIRECTION('ref_axis',(0.999999974259828,-0.000226892800803726,0.));
#30292=DIRECTION('center_axis',(0.,0.,1.));
#30293=DIRECTION('ref_axis',(0.999999974259828,-0.000226892800803726,0.));
#30294=DIRECTION('',(0.,0.,1.));
#30295=DIRECTION('center_axis',(0.999999974259828,-0.000226892800803133,
0.));
#30296=DIRECTION('ref_axis',(0.000226892800803133,0.999999974259828,0.));
#30297=DIRECTION('',(0.000226892800803133,0.999999974259828,0.));
#30298=DIRECTION('',(0.,0.,1.));
#30299=DIRECTION('center_axis',(0.,0.,1.));
#30300=DIRECTION('ref_axis',(-0.999999974259828,0.000226892800803038,0.));
#30301=DIRECTION('center_axis',(0.,0.,-1.));
#30302=DIRECTION('ref_axis',(-0.999999974259828,0.000226892800803038,0.));
#30303=DIRECTION('',(0.,0.,1.));
#30304=DIRECTION('center_axis',(0.320612990585676,0.947210277746029,0.));
#30305=DIRECTION('ref_axis',(-0.947210277746029,0.320612990585676,0.));
#30306=DIRECTION('',(-0.947210277746029,0.320612990585676,0.));
#30307=DIRECTION('',(0.,0.,1.));
#30308=DIRECTION('center_axis',(0.123601476740492,-0.992331937885489,0.));
#30309=DIRECTION('ref_axis',(0.992331937885489,0.123601476740492,0.));
#30310=DIRECTION('',(0.992331937885489,0.123601476740492,0.));
#30311=DIRECTION('',(0.,0.,1.));
#30312=DIRECTION('center_axis',(0.,-1.,0.));
#30313=DIRECTION('ref_axis',(1.,0.,0.));
#30314=DIRECTION('',(1.,0.,0.));
#30315=DIRECTION('center_axis',(0.,0.,1.));
#30316=DIRECTION('ref_axis',(1.,0.,0.));
#35982=CARTESIAN_POINT('',(0.,0.,0.));
#35983=CARTESIAN_POINT('Origin',(0.,18.7095,-22.));
#35984=CARTESIAN_POINT('',(2.0145,16.8045,-22.));
#35985=CARTESIAN_POINT('',(-2.0145,16.8045,-22.));
#35986=CARTESIAN_POINT('',(-2.0145,16.8045,-22.));
#35987=CARTESIAN_POINT('',(-4.76226713600492,17.1467524890944,-22.));
#35988=CARTESIAN_POINT('',(-2.0145,16.8045,-22.));
#35989=CARTESIAN_POINT('',(-2.86121610856864,17.7902227611999,-22.));
#35990=CARTESIAN_POINT('',(-4.76226713600492,17.1467524890944,-22.));
#35991=CARTESIAN_POINT('',(-2.77493396164202,17.9105472818593,-22.));
#35992=CARTESIAN_POINT('Origin',(-2.90193395837302,17.9105184664736,-22.));
#35993=CARTESIAN_POINT('',(-2.77524548545753,19.2835472465181,-22.));
#35994=CARTESIAN_POINT('',(-2.77493396164202,17.9105472818593,-22.));
#35995=CARTESIAN_POINT('',(-2.50285868490141,19.4743666560534,-22.));
#35996=CARTESIAN_POINT('Origin',(-2.57224549068278,19.2835933057566,-22.));
#35997=CARTESIAN_POINT('',(-1.1157578719061,18.9698596347071,-22.));
#35998=CARTESIAN_POINT('',(-2.50285868490141,19.4743666560534,-22.));
#35999=CARTESIAN_POINT('',(-1.06752374914854,18.9384317981151,-22.));
#36000=CARTESIAN_POINT('Origin',(-1.15916735138508,18.8505088194968,-22.));
#36001=CARTESIAN_POINT('',(-0.749754873669872,18.6072159443625,-22.));
#36002=CARTESIAN_POINT('',(-1.06752374914854,18.9384317981151,-22.));
#36003=CARTESIAN_POINT('',(-0.476019974175079,18.7173288203203,-22.));
#36004=CARTESIAN_POINT('Origin',(-0.635019970082392,18.7172927443649,-22.));
#36005=CARTESIAN_POINT('',(-0.476404103686861,20.4103287767422,-22.));
#36006=CARTESIAN_POINT('',(-0.476019974175079,18.7173288203203,-22.));
#36007=CARTESIAN_POINT('',(-0.27345016815068,20.6133748307555,-22.));
#36008=CARTESIAN_POINT('Origin',(-0.273404108912115,20.4103748359807,-22.));
#36009=CARTESIAN_POINT('',(0.,20.6145,-22.));
#36010=CARTESIAN_POINT('',(-0.27345016815068,20.6133748307555,-22.));
#36011=CARTESIAN_POINT('',(0.27345016815068,20.6133748307555,-22.));
#36012=CARTESIAN_POINT('',(0.27345016815068,20.6133748307555,-22.));
#36013=CARTESIAN_POINT('',(0.47640410368686,20.4103287767422,-22.));
#36014=CARTESIAN_POINT('Origin',(0.273404108912115,20.4103748359807,-22.));
#36015=CARTESIAN_POINT('',(0.476019974175079,18.7173288203203,-22.));
#36016=CARTESIAN_POINT('',(0.476019974175079,18.7173288203203,-22.));
#36017=CARTESIAN_POINT('',(0.749754873669872,18.6072159443625,-22.));
#36018=CARTESIAN_POINT('Origin',(0.635019970082392,18.7172927443649,-22.));
#36019=CARTESIAN_POINT('',(1.06752374914854,18.9384317981151,-22.));
#36020=CARTESIAN_POINT('',(1.06752374914854,18.9384317981151,-22.));
#36021=CARTESIAN_POINT('',(1.1157578719061,18.9698596347071,-22.));
#36022=CARTESIAN_POINT('Origin',(1.15916735138508,18.8505088194968,-22.));
#36023=CARTESIAN_POINT('',(2.50285868490141,19.4743666560534,-22.));
#36024=CARTESIAN_POINT('',(2.50285868490141,19.4743666560534,-22.));
#36025=CARTESIAN_POINT('',(2.77524548545753,19.2835472465181,-22.));
#36026=CARTESIAN_POINT('Origin',(2.57224549068278,19.2835933057566,-22.));
#36027=CARTESIAN_POINT('',(2.77493396164202,17.9105472818593,-22.));
#36028=CARTESIAN_POINT('',(2.77493396164202,17.9105472818593,-22.));
#36029=CARTESIAN_POINT('',(2.86121610856864,17.7902227611999,-22.));
#36030=CARTESIAN_POINT('Origin',(2.90193395837302,17.9105184664736,-22.));
#36031=CARTESIAN_POINT('',(4.76226713600492,17.1467524890944,-22.));
#36032=CARTESIAN_POINT('',(4.76226713600492,17.1467524890944,-22.));
#36033=CARTESIAN_POINT('',(2.0145,16.8045,-22.));
#36034=CARTESIAN_POINT('Origin',(-4.76226713600492,17.1467524890944,0.));
#36035=CARTESIAN_POINT('',(-2.0145,16.8045,422.));
#36036=CARTESIAN_POINT('',(-2.0145,16.8045,0.));
#36037=CARTESIAN_POINT('',(-4.76226713600492,17.1467524890944,422.));
#36038=CARTESIAN_POINT('',(-2.0145,16.8045,422.));
#36039=CARTESIAN_POINT('',(-4.76226713600492,17.1467524890944,0.));
#36040=CARTESIAN_POINT('Origin',(-2.86121610856864,17.7902227611999,0.));
#36041=CARTESIAN_POINT('',(-2.86121610856864,17.7902227611999,422.));
#36042=CARTESIAN_POINT('',(-4.76226713600492,17.1467524890944,422.));
#36043=CARTESIAN_POINT('',(-2.86121610856864,17.7902227611999,0.));
#36044=CARTESIAN_POINT('Origin',(-2.90193395837302,17.9105184664736,0.));
#36045=CARTESIAN_POINT('',(-2.77493396164202,17.9105472818593,422.));
#36046=CARTESIAN_POINT('Origin',(-2.90193395837302,17.9105184664736,422.));
#36047=CARTESIAN_POINT('',(-2.77493396164202,17.9105472818593,0.));
#36048=CARTESIAN_POINT('Origin',(-2.77524548545753,19.2835472465181,0.));
#36049=CARTESIAN_POINT('',(-2.77524548545753,19.2835472465181,422.));
#36050=CARTESIAN_POINT('',(-2.77493396164202,17.9105472818593,422.));
#36051=CARTESIAN_POINT('',(-2.77524548545753,19.2835472465181,0.));
#36052=CARTESIAN_POINT('Origin',(-2.57224549068278,19.2835933057566,0.));
#36053=CARTESIAN_POINT('',(-2.50285868490141,19.4743666560534,422.));
#36054=CARTESIAN_POINT('Origin',(-2.57224549068278,19.2835933057566,422.));
#36055=CARTESIAN_POINT('',(-2.50285868490141,19.4743666560534,0.));
#36056=CARTESIAN_POINT('Origin',(-1.1157578719061,18.9698596347071,0.));
#36057=CARTESIAN_POINT('',(-1.1157578719061,18.9698596347071,422.));
#36058=CARTESIAN_POINT('',(-2.50285868490141,19.4743666560534,422.));
#36059=CARTESIAN_POINT('',(-1.1157578719061,18.9698596347071,0.));
#36060=CARTESIAN_POINT('Origin',(-1.15916735138508,18.8505088194968,0.));
#36061=CARTESIAN_POINT('',(-1.06752374914854,18.9384317981151,422.));
#36062=CARTESIAN_POINT('Origin',(-1.15916735138508,18.8505088194968,422.));
#36063=CARTESIAN_POINT('',(-1.06752374914854,18.9384317981151,0.));
#36064=CARTESIAN_POINT('Origin',(-0.749754873669872,18.6072159443625,0.));
#36065=CARTESIAN_POINT('',(-0.749754873669872,18.6072159443625,422.));
#36066=CARTESIAN_POINT('',(-1.06752374914854,18.9384317981151,422.));
#36067=CARTESIAN_POINT('',(-0.749754873669872,18.6072159443625,0.));
#36068=CARTESIAN_POINT('Origin',(-0.635019970082392,18.7172927443649,0.));
#36069=CARTESIAN_POINT('',(-0.476019974175079,18.7173288203203,422.));
#36070=CARTESIAN_POINT('Origin',(-0.635019970082392,18.7172927443649,422.));
#36071=CARTESIAN_POINT('',(-0.476019974175079,18.7173288203203,0.));
#36072=CARTESIAN_POINT('Origin',(-0.47640410368686,20.4103287767422,0.));
#36073=CARTESIAN_POINT('',(-0.476404103686861,20.4103287767422,422.));
#36074=CARTESIAN_POINT('',(-0.476019974175079,18.7173288203203,422.));
#36075=CARTESIAN_POINT('',(-0.476404103686861,20.4103287767422,0.));
#36076=CARTESIAN_POINT('Origin',(-0.273404108912115,20.4103748359807,0.));
#36077=CARTESIAN_POINT('',(-0.27345016815068,20.6133748307555,422.));
#36078=CARTESIAN_POINT('Origin',(-0.273404108912115,20.4103748359807,422.));
#36079=CARTESIAN_POINT('',(-0.27345016815068,20.6133748307555,0.));
#36080=CARTESIAN_POINT('Origin',(0.,20.6145,0.));
#36081=CARTESIAN_POINT('',(0.,20.6145,422.));
#36082=CARTESIAN_POINT('',(-0.27345016815068,20.6133748307555,422.));
#36083=CARTESIAN_POINT('',(0.,20.6145,0.));
#36084=CARTESIAN_POINT('Origin',(0.27345016815068,20.6133748307555,0.));
#36085=CARTESIAN_POINT('',(0.27345016815068,20.6133748307555,422.));
#36086=CARTESIAN_POINT('',(0.27345016815068,20.6133748307555,422.));
#36087=CARTESIAN_POINT('',(0.27345016815068,20.6133748307555,0.));
#36088=CARTESIAN_POINT('Origin',(0.273404108912115,20.4103748359807,0.));
#36089=CARTESIAN_POINT('',(0.47640410368686,20.4103287767422,422.));
#36090=CARTESIAN_POINT('Origin',(0.273404108912115,20.4103748359807,422.));
#36091=CARTESIAN_POINT('',(0.47640410368686,20.4103287767422,0.));
#36092=CARTESIAN_POINT('Origin',(0.476019974175079,18.7173288203203,0.));
#36093=CARTESIAN_POINT('',(0.476019974175079,18.7173288203203,422.));
#36094=CARTESIAN_POINT('',(0.476019974175079,18.7173288203203,422.));
#36095=CARTESIAN_POINT('',(0.476019974175079,18.7173288203203,0.));
#36096=CARTESIAN_POINT('Origin',(0.635019970082392,18.7172927443649,0.));
#36097=CARTESIAN_POINT('',(0.749754873669872,18.6072159443625,422.));
#36098=CARTESIAN_POINT('Origin',(0.635019970082392,18.7172927443649,422.));
#36099=CARTESIAN_POINT('',(0.749754873669872,18.6072159443625,0.));
#36100=CARTESIAN_POINT('Origin',(1.06752374914854,18.9384317981151,0.));
#36101=CARTESIAN_POINT('',(1.06752374914854,18.9384317981151,422.));
#36102=CARTESIAN_POINT('',(1.06752374914854,18.9384317981151,422.));
#36103=CARTESIAN_POINT('',(1.06752374914854,18.9384317981151,0.));
#36104=CARTESIAN_POINT('Origin',(1.15916735138508,18.8505088194968,0.));
#36105=CARTESIAN_POINT('',(1.1157578719061,18.9698596347071,422.));
#36106=CARTESIAN_POINT('Origin',(1.15916735138508,18.8505088194968,422.));
#36107=CARTESIAN_POINT('',(1.1157578719061,18.9698596347071,0.));
#36108=CARTESIAN_POINT('Origin',(2.50285868490141,19.4743666560534,0.));
#36109=CARTESIAN_POINT('',(2.50285868490141,19.4743666560534,422.));
#36110=CARTESIAN_POINT('',(2.50285868490141,19.4743666560534,422.));
#36111=CARTESIAN_POINT('',(2.50285868490141,19.4743666560534,0.));
#36112=CARTESIAN_POINT('Origin',(2.57224549068278,19.2835933057566,0.));
#36113=CARTESIAN_POINT('',(2.77524548545753,19.2835472465181,422.));
#36114=CARTESIAN_POINT('Origin',(2.57224549068278,19.2835933057566,422.));
#36115=CARTESIAN_POINT('',(2.77524548545753,19.2835472465181,0.));
#36116=CARTESIAN_POINT('Origin',(2.77493396164202,17.9105472818593,0.));
#36117=CARTESIAN_POINT('',(2.77493396164202,17.9105472818593,422.));
#36118=CARTESIAN_POINT('',(2.77493396164202,17.9105472818593,422.));
#36119=CARTESIAN_POINT('',(2.77493396164202,17.9105472818593,0.));
#36120=CARTESIAN_POINT('Origin',(2.90193395837302,17.9105184664736,0.));
#36121=CARTESIAN_POINT('',(2.86121610856864,17.7902227611999,422.));
#36122=CARTESIAN_POINT('Origin',(2.90193395837302,17.9105184664736,422.));
#36123=CARTESIAN_POINT('',(2.86121610856864,17.7902227611999,0.));
#36124=CARTESIAN_POINT('Origin',(4.76226713600492,17.1467524890944,0.));
#36125=CARTESIAN_POINT('',(4.76226713600492,17.1467524890944,422.));
#36126=CARTESIAN_POINT('',(4.76226713600492,17.1467524890944,422.));
#36127=CARTESIAN_POINT('',(4.76226713600492,17.1467524890944,0.));
#36128=CARTESIAN_POINT('Origin',(2.0145,16.8045,0.));
#36129=CARTESIAN_POINT('',(2.0145,16.8045,422.));
#36130=CARTESIAN_POINT('',(2.0145,16.8045,422.));
#36131=CARTESIAN_POINT('',(2.0145,16.8045,0.));
#36132=CARTESIAN_POINT('Origin',(-2.0145,16.8045,0.));
#36133=CARTESIAN_POINT('',(-2.0145,16.8045,422.));
#36134=CARTESIAN_POINT('Origin',(0.,18.7095,422.));
#215589=UNCERTAINTY_MEASURE_WITH_UNIT(LENGTH_MEASURE(0.01),#215610,
'DISTANCE_ACCURACY_VALUE',
'Maximum model space distance between geometric entities at asserted c
onnectivities');
#215598=UNCERTAINTY_MEASURE_WITH_UNIT(LENGTH_MEASURE(0.01),#215610,
'DISTANCE_ACCURACY_VALUE',
'Maximum model space distance between geometric entities at asserted c
onnectivities');
#215600=(
GEOMETRIC_REPRESENTATION_CONTEXT(3)
GLOBAL_UNCERTAINTY_ASSIGNED_CONTEXT((#215589))
GLOBAL_UNIT_ASSIGNED_CONTEXT((#215610,#215612,#215613))
REPRESENTATION_CONTEXT('','3D')
);
#215609=(
GEOMETRIC_REPRESENTATION_CONTEXT(3)
GLOBAL_UNCERTAINTY_ASSIGNED_CONTEXT((#215598))
GLOBAL_UNIT_ASSIGNED_CONTEXT((#215610,#215612,#215613))
REPRESENTATION_CONTEXT('','3D')
);
#215610=(
LENGTH_UNIT()
NAMED_UNIT(*)
SI_UNIT(.MILLI.,.METRE.)
);
#215612=(
NAMED_UNIT(*)
PLANE_ANGLE_UNIT()
SI_UNIT($,.RADIAN.)
);
#215613=(
NAMED_UNIT(*)
SI_UNIT($,.STERADIAN.)
SOLID_ANGLE_UNIT()
);
#215615=SHAPE_DEFINITION_REPRESENTATION(#215625,#215644);
#215625=PRODUCT_DEFINITION_SHAPE('',$,#215655);
#215644=SHAPE_REPRESENTATION('',(#28179),#215600);
#215653=PRODUCT_DEFINITION_CONTEXT('part definition',#215685,'design');
#215655=PRODUCT_DEFINITION('2026-10-04-09-58-43-959','TopStrip',#215665,
#215653);
#215665=PRODUCT_DEFINITION_FORMATION('',$,#215688);
#215685=APPLICATION_CONTEXT(
'Core Data for Automotive Mechanical Design Process');
#215686=PRODUCT_CONTEXT('part definition',#215685,'mechanical');
#215688=PRODUCT('2026-10-04-09-58-43-959','TopStrip',$,(#215686));
#215698=PRESENTATION_STYLE_ASSIGNMENT((#215700));
#215700=SURFACE_STYLE_USAGE(.BOTH.,#215702);
#215702=SURFACE_SIDE_STYLE('',(#215704));
#215704=SURFACE_STYLE_FILL_AREA(#215706);
#215706=FILL_AREA_STYLE('Opaque(245,245,246)',(#215708));
#215708=FILL_AREA_STYLE_COLOUR('Opaque(245,245,246)',#215710);
#215710=COLOUR_RGB('Opaque(245,245,246)', 0.66274510, 0.83137255, 0.94901961);
ENDSEC;
END-ISO-10303-21;
